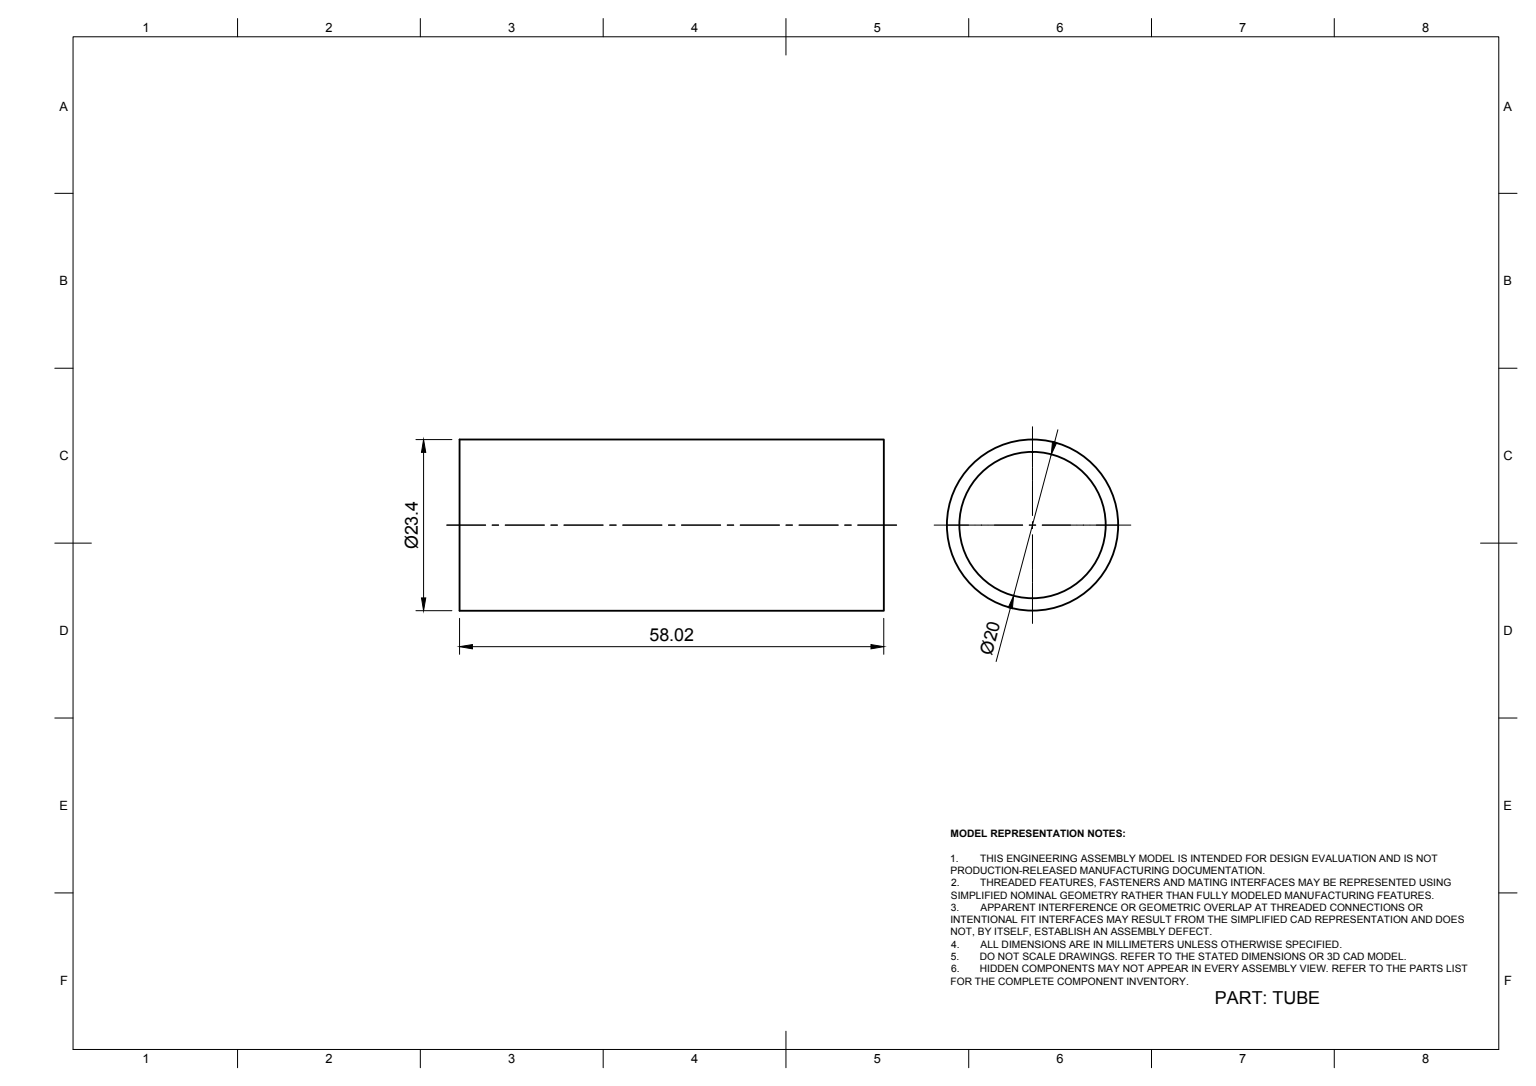
ISO-10303-21;
HEADER;
/* Generated by software containing ST-Developer
 * from STEP Tools, Inc. (www.steptools.com) 
 */

FILE_DESCRIPTION(
/* description */ (''),
/* implementation_level */ '2;1');

FILE_NAME(
/* name */ 'Tube.step',
/* time_stamp */ '2026-10-04T22:56:18-07:00',
/* author */ (''),
/* organization */ (''),
/* preprocessor_version */ 'ST-DEVELOPER v20.2',
/* originating_system */ 'Autodesk Translation Framework v15.15.0.0',
/* authorisation */ '');

FILE_SCHEMA (('AUTOMOTIVE_DESIGN { 1 0 10303 214 3 1 1 }'));
ENDSEC;

DATA;
#10=MECHANICAL_DESIGN_GEOMETRIC_PRESENTATION_REPRESENTATION('',(#190),#14544);
#174=SHAPE_REPRESENTATION_RELATIONSHIP('SRR','None',#14576,#182);
#182=ADVANCED_BREP_SHAPE_REPRESENTATION('',(#198),#14536);
#190=STYLED_ITEM('',(#14625),#198);
#198=MANIFOLD_SOLID_BREP('Body1',#1826);
#206=LINE('',#2607,#262);
#207=LINE('',#2609,#263);
#262=VECTOR('',#2146,10.0021025234003);
#263=VECTOR('',#2149,11.7021025234003);
#318=CYLINDRICAL_SURFACE('',#1931,10.0021025234003);
#319=CYLINDRICAL_SURFACE('',#1932,11.7021025234003);
#370=FACE_BOUND('',#505,.T.);
#371=FACE_BOUND('',#507,.T.);
#399=FACE_OUTER_BOUND('',#504,.T.);
#400=FACE_OUTER_BOUND('',#506,.T.);
#401=FACE_OUTER_BOUND('',#508,.T.);
#402=FACE_OUTER_BOUND('',#509,.T.);
#504=EDGE_LOOP('',(#1171));
#505=EDGE_LOOP('',(#1172));
#506=EDGE_LOOP('',(#1173));
#507=EDGE_LOOP('',(#1174));
#508=EDGE_LOOP('',(#1175,#1176,#1177,#1178));
#509=EDGE_LOOP('',(#1179,#1180,#1181,#1182));
#638=CIRCLE('',#1926,11.7021025234003);
#639=CIRCLE('',#1927,10.0021025234003);
#640=CIRCLE('',#1929,11.7021025234003);
#641=CIRCLE('',#1930,10.0021025234003);
#725=VERTEX_POINT('',#2597);
#726=VERTEX_POINT('',#2599);
#727=VERTEX_POINT('',#2602);
#728=VERTEX_POINT('',#2604);
#914=EDGE_CURVE('',#725,#725,#638,.T.);
#915=EDGE_CURVE('',#726,#726,#639,.T.);
#916=EDGE_CURVE('',#727,#727,#640,.T.);
#917=EDGE_CURVE('',#728,#728,#641,.T.);
#918=EDGE_CURVE('',#728,#726,#206,.T.);
#919=EDGE_CURVE('',#725,#727,#207,.T.);
#1171=ORIENTED_EDGE('',*,*,#914,.T.);
#1172=ORIENTED_EDGE('',*,*,#915,.F.);
#1173=ORIENTED_EDGE('',*,*,#916,.F.);
#1174=ORIENTED_EDGE('',*,*,#917,.T.);
#1175=ORIENTED_EDGE('',*,*,#917,.F.);
#1176=ORIENTED_EDGE('',*,*,#918,.T.);
#1177=ORIENTED_EDGE('',*,*,#915,.T.);
#1178=ORIENTED_EDGE('',*,*,#918,.F.);
#1179=ORIENTED_EDGE('',*,*,#914,.F.);
#1180=ORIENTED_EDGE('',*,*,#919,.T.);
#1181=ORIENTED_EDGE('',*,*,#916,.T.);
#1182=ORIENTED_EDGE('',*,*,#919,.F.);
#1685=PLANE('',#1925);
#1686=PLANE('',#1928);
#1721=ADVANCED_FACE('',(#399,#370),#1685,.T.);
#1722=ADVANCED_FACE('',(#400,#371),#1686,.T.);
#1723=ADVANCED_FACE('',(#401),#318,.F.);
#1724=ADVANCED_FACE('',(#402),#319,.T.);
#1826=CLOSED_SHELL('',(#1721,#1722,#1723,#1724));
#1924=AXIS2_PLACEMENT_3D('',#2595,#2130,#2131);
#1925=AXIS2_PLACEMENT_3D('',#2596,#2132,#2133);
#1926=AXIS2_PLACEMENT_3D('',#2598,#2134,#2135);
#1927=AXIS2_PLACEMENT_3D('',#2600,#2136,#2137);
#1928=AXIS2_PLACEMENT_3D('',#2601,#2138,#2139);
#1929=AXIS2_PLACEMENT_3D('',#2603,#2140,#2141);
#1930=AXIS2_PLACEMENT_3D('',#2605,#2142,#2143);
#1931=AXIS2_PLACEMENT_3D('',#2606,#2144,#2145);
#1932=AXIS2_PLACEMENT_3D('',#2608,#2147,#2148);
#2130=DIRECTION('axis',(0.,0.,1.));
#2131=DIRECTION('refdir',(1.,0.,0.));
#2132=DIRECTION('center_axis',(0.,0.,1.));
#2133=DIRECTION('ref_axis',(1.,0.,0.));
#2134=DIRECTION('center_axis',(0.,0.,1.));
#2135=DIRECTION('ref_axis',(1.,0.,0.));
#2136=DIRECTION('center_axis',(0.,0.,1.));
#2137=DIRECTION('ref_axis',(1.,0.,0.));
#2138=DIRECTION('center_axis',(0.,0.,-1.));
#2139=DIRECTION('ref_axis',(-1.,0.,0.));
#2140=DIRECTION('center_axis',(0.,0.,1.));
#2141=DIRECTION('ref_axis',(1.,0.,0.));
#2142=DIRECTION('center_axis',(0.,0.,1.));
#2143=DIRECTION('ref_axis',(1.,0.,0.));
#2144=DIRECTION('center_axis',(0.,0.,1.));
#2145=DIRECTION('ref_axis',(1.,0.,0.));
#2146=DIRECTION('',(0.,0.,1.));
#2147=DIRECTION('center_axis',(0.,0.,1.));
#2148=DIRECTION('ref_axis',(1.,0.,0.));
#2149=DIRECTION('',(0.,0.,-1.));
#2595=CARTESIAN_POINT('',(0.,0.,0.));
#2596=CARTESIAN_POINT('Origin',(10.0021025234003,0.,86.3550920810876));
#2597=CARTESIAN_POINT('',(-11.7021025234003,-1.43309423985764E-15,86.3550920810876));
#2598=CARTESIAN_POINT('Origin',(0.,0.,86.3550920810876));
#2599=CARTESIAN_POINT('',(-10.0021025234003,-1.22490428400259E-15,86.3550920810876));
#2600=CARTESIAN_POINT('Origin',(0.,0.,86.3550920810876));
#2601=CARTESIAN_POINT('Origin',(11.7021025234003,0.,28.3343056886915));
#2602=CARTESIAN_POINT('',(-11.7021025234003,-1.43309423985764E-15,28.3343056886915));
#2603=CARTESIAN_POINT('Origin',(0.,0.,28.3343056886915));
#2604=CARTESIAN_POINT('',(-10.0021025234003,-1.22490428400259E-15,28.3343056886915));
#2605=CARTESIAN_POINT('Origin',(0.,0.,28.3343056886915));
#2606=CARTESIAN_POINT('Origin',(0.,0.,52.3446988848895));
#2607=CARTESIAN_POINT('',(-10.0021025234003,-1.22490428400258E-15,52.3446988848895));
#2608=CARTESIAN_POINT('Origin',(0.,0.,52.3446988848895));
#2609=CARTESIAN_POINT('',(-11.7021025234003,-1.43309423985763E-15,52.3446988848895));
#14526=UNCERTAINTY_MEASURE_WITH_UNIT(LENGTH_MEASURE(0.01),#14545,
'DISTANCE_ACCURACY_VALUE',
'Maximum model space distance between geometric entities at asserted c
onnectivities');
#14534=UNCERTAINTY_MEASURE_WITH_UNIT(LENGTH_MEASURE(0.01),#14545,
'DISTANCE_ACCURACY_VALUE',
'Maximum model space distance between geometric entities at asserted c
onnectivities');
#14536=(
GEOMETRIC_REPRESENTATION_CONTEXT(3)
GLOBAL_UNCERTAINTY_ASSIGNED_CONTEXT((#14526))
GLOBAL_UNIT_ASSIGNED_CONTEXT((#14545,#14547,#14548))
REPRESENTATION_CONTEXT('','3D')
);
#14544=(
GEOMETRIC_REPRESENTATION_CONTEXT(3)
GLOBAL_UNCERTAINTY_ASSIGNED_CONTEXT((#14534))
GLOBAL_UNIT_ASSIGNED_CONTEXT((#14545,#14547,#14548))
REPRESENTATION_CONTEXT('','3D')
);
#14545=(
LENGTH_UNIT()
NAMED_UNIT(*)
SI_UNIT(.MILLI.,.METRE.)
);
#14547=(
NAMED_UNIT(*)
PLANE_ANGLE_UNIT()
SI_UNIT($,.RADIAN.)
);
#14548=(
NAMED_UNIT(*)
SI_UNIT($,.STERADIAN.)
SOLID_ANGLE_UNIT()
);
#14550=SHAPE_DEFINITION_REPRESENTATION(#14559,#14576);
#14559=PRODUCT_DEFINITION_SHAPE('',$,#14586);
#14576=SHAPE_REPRESENTATION('',(#1924),#14536);
#14584=PRODUCT_DEFINITION_CONTEXT('part definition',#14613,'design');
#14586=PRODUCT_DEFINITION('Tube','Tube',#14595,#14584);
#14595=PRODUCT_DEFINITION_FORMATION('',$,#14616);
#14613=APPLICATION_CONTEXT(
'Core Data for Automotive Mechanical Design Process');
#14614=PRODUCT_CONTEXT('part definition',#14613,'mechanical');
#14616=PRODUCT('Tube','Tube',$,(#14614));
#14625=PRESENTATION_STYLE_ASSIGNMENT((#14629));
#14629=SURFACE_STYLE_USAGE(.BOTH.,#14633);
#14633=SURFACE_SIDE_STYLE('',(#14637));
#14637=SURFACE_STYLE_FILL_AREA(#14641);
#14641=FILL_AREA_STYLE('Opaque(246,246,243)',(#14645));
#14645=FILL_AREA_STYLE_COLOUR('Opaque(246,246,243)',#14649);
#14649=COLOUR_RGB('Opaque(246,246,243)', 0.09019608, 0.27058824, 0.51372549);
ENDSEC;
END-ISO-10303-21;
